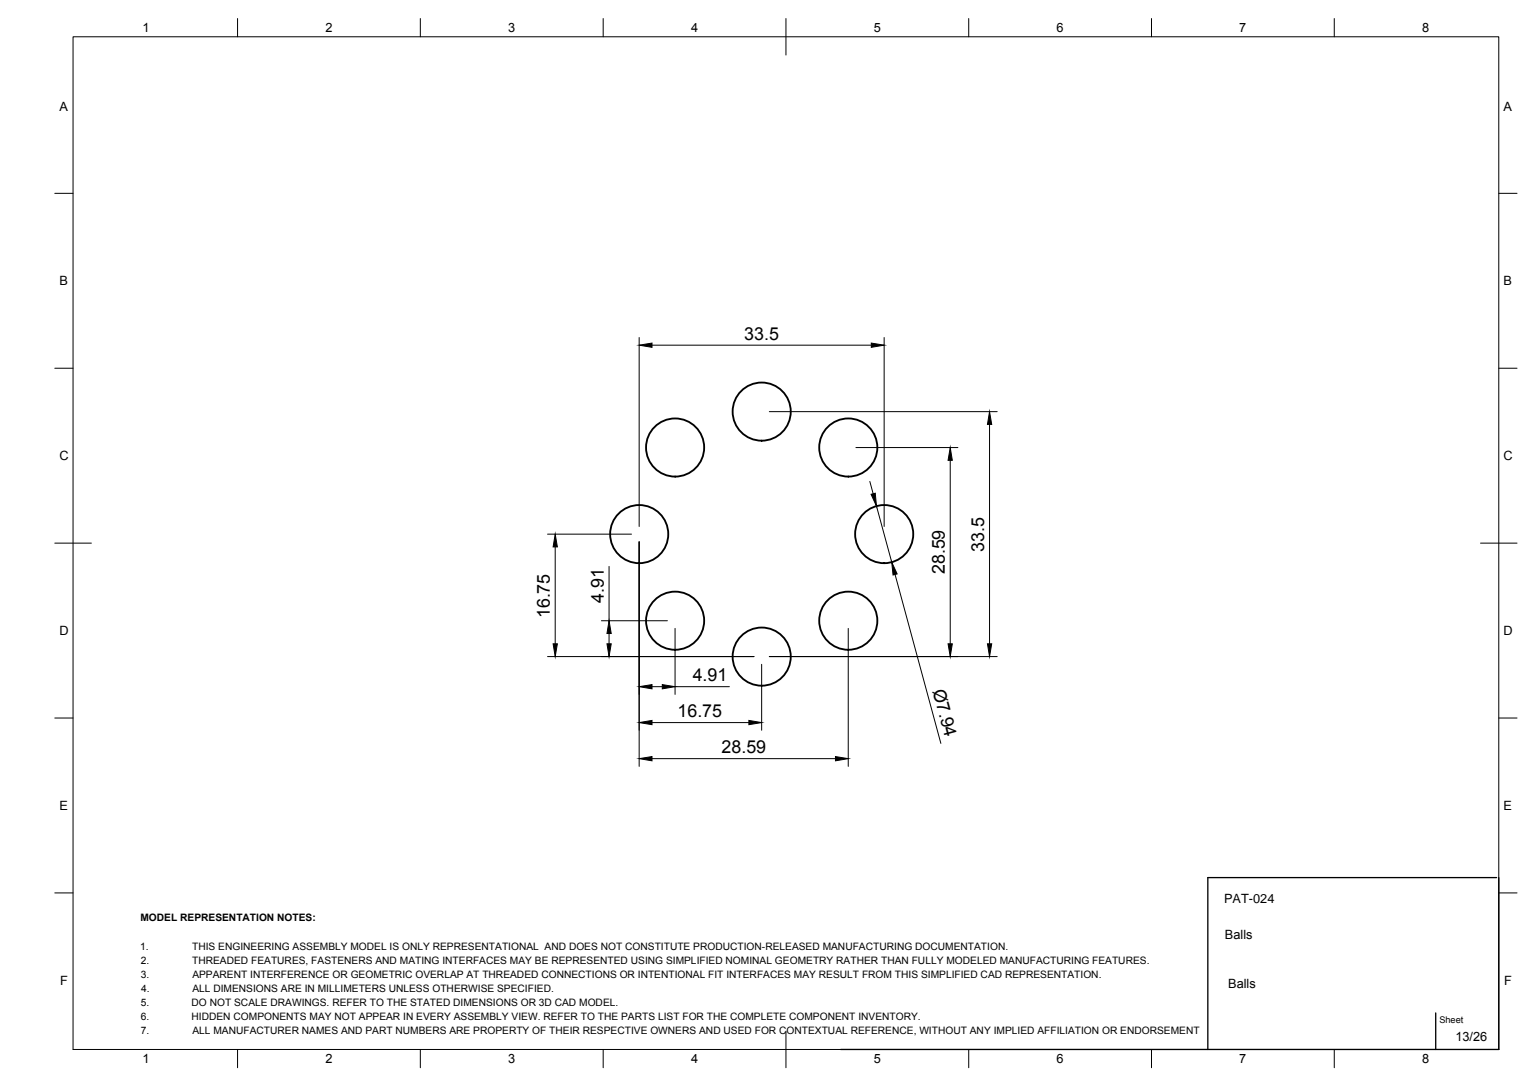
ISO-10303-21;
HEADER;
/* Generated by software containing ST-Developer
 * from STEP Tools, Inc. (www.steptools.com) 
 */

FILE_DESCRIPTION(
/* description */ ('Compact handwheel screw vise'),
/* implementation_level */ '2;1');

FILE_NAME(
/* name */ 'Balls.step',
/* time_stamp */ '2026-10-29T16:08:22-07:00',
/* author */ (''),
/* organization */ (''),
/* preprocessor_version */ 'ST-DEVELOPER v20.2',
/* originating_system */ 'Autodesk Translation Framework v15.17.0.0',
/* authorisation */ '');

FILE_SCHEMA (('AUTOMOTIVE_DESIGN { 1 0 10303 214 3 1 1 }'));
ENDSEC;

DATA;
#10=MECHANICAL_DESIGN_GEOMETRIC_PRESENTATION_REPRESENTATION('',(#653,#654,#655,#656,#657,#658,#659,#660),#25074);
#541=SPHERICAL_SURFACE('',#8614,0.3969);
#542=SPHERICAL_SURFACE('',#8616,0.3969);
#543=SPHERICAL_SURFACE('',#8618,0.3969);
#544=SPHERICAL_SURFACE('',#8620,0.3969);
#545=SPHERICAL_SURFACE('',#8622,0.3969);
#546=SPHERICAL_SURFACE('',#8624,0.3969);
#547=SPHERICAL_SURFACE('',#8626,0.3969);
#548=SPHERICAL_SURFACE('',#8628,0.3969);
#597=SHAPE_REPRESENTATION_RELATIONSHIP('SRR','None',#25206,#625);
#625=ADVANCED_BREP_SHAPE_REPRESENTATION('',(#688,#689,#690,#691,#692,#693,
#694,#695),#25053);
#653=STYLED_ITEM('',(#25439),#688);
#654=STYLED_ITEM('',(#25439),#689);
#655=STYLED_ITEM('',(#25439),#690);
#656=STYLED_ITEM('',(#25439),#691);
#657=STYLED_ITEM('',(#25439),#692);
#658=STYLED_ITEM('',(#25439),#693);
#659=STYLED_ITEM('',(#25439),#694);
#660=STYLED_ITEM('',(#25439),#695);
#688=MANIFOLD_SOLID_BREP('Body1',#8062);
#689=MANIFOLD_SOLID_BREP('Body2',#8063);
#690=MANIFOLD_SOLID_BREP('Body3',#8064);
#691=MANIFOLD_SOLID_BREP('Body4',#8065);
#692=MANIFOLD_SOLID_BREP('Body5',#8066);
#693=MANIFOLD_SOLID_BREP('Body6',#8067);
#694=MANIFOLD_SOLID_BREP('Body7',#8068);
#695=MANIFOLD_SOLID_BREP('Body8',#8069);
#1121=FACE_OUTER_BOUND('',#1643,.T.);
#1122=FACE_OUTER_BOUND('',#1644,.T.);
#1123=FACE_OUTER_BOUND('',#1645,.T.);
#1124=FACE_OUTER_BOUND('',#1646,.T.);
#1125=FACE_OUTER_BOUND('',#1647,.T.);
#1126=FACE_OUTER_BOUND('',#1648,.T.);
#1127=FACE_OUTER_BOUND('',#1649,.T.);
#1128=FACE_OUTER_BOUND('',#1650,.T.);
#1643=EDGE_LOOP('',(#5595,#5596));
#1644=EDGE_LOOP('',(#5597,#5598));
#1645=EDGE_LOOP('',(#5599,#5600));
#1646=EDGE_LOOP('',(#5601,#5602));
#1647=EDGE_LOOP('',(#5603,#5604));
#1648=EDGE_LOOP('',(#5605,#5606));
#1649=EDGE_LOOP('',(#5607,#5608));
#1650=EDGE_LOOP('',(#5609,#5610));
#3169=CIRCLE('',#8615,0.3969);
#3170=CIRCLE('',#8617,0.3969);
#3171=CIRCLE('',#8619,0.3969);
#3172=CIRCLE('',#8621,0.3969);
#3173=CIRCLE('',#8623,0.3969);
#3174=CIRCLE('',#8625,0.3969);
#3175=CIRCLE('',#8627,0.3969);
#3176=CIRCLE('',#8629,0.3969);
#3476=VERTEX_POINT('',#11802);
#3477=VERTEX_POINT('',#11803);
#3478=VERTEX_POINT('',#11806);
#3479=VERTEX_POINT('',#11807);
#3480=VERTEX_POINT('',#11810);
#3481=VERTEX_POINT('',#11811);
#3482=VERTEX_POINT('',#11814);
#3483=VERTEX_POINT('',#11815);
#3484=VERTEX_POINT('',#11818);
#3485=VERTEX_POINT('',#11819);
#3486=VERTEX_POINT('',#11822);
#3487=VERTEX_POINT('',#11823);
#3488=VERTEX_POINT('',#11826);
#3489=VERTEX_POINT('',#11827);
#3490=VERTEX_POINT('',#11830);
#3491=VERTEX_POINT('',#11831);
#4284=EDGE_CURVE('',#3476,#3477,#3169,.T.);
#4285=EDGE_CURVE('',#3478,#3479,#3170,.T.);
#4286=EDGE_CURVE('',#3480,#3481,#3171,.T.);
#4287=EDGE_CURVE('',#3482,#3483,#3172,.T.);
#4288=EDGE_CURVE('',#3484,#3485,#3173,.T.);
#4289=EDGE_CURVE('',#3486,#3487,#3174,.T.);
#4290=EDGE_CURVE('',#3488,#3489,#3175,.T.);
#4291=EDGE_CURVE('',#3490,#3491,#3176,.T.);
#5595=ORIENTED_EDGE('',*,*,#4284,.T.);
#5596=ORIENTED_EDGE('',*,*,#4284,.F.);
#5597=ORIENTED_EDGE('',*,*,#4285,.T.);
#5598=ORIENTED_EDGE('',*,*,#4285,.F.);
#5599=ORIENTED_EDGE('',*,*,#4286,.T.);
#5600=ORIENTED_EDGE('',*,*,#4286,.F.);
#5601=ORIENTED_EDGE('',*,*,#4287,.T.);
#5602=ORIENTED_EDGE('',*,*,#4287,.F.);
#5603=ORIENTED_EDGE('',*,*,#4288,.T.);
#5604=ORIENTED_EDGE('',*,*,#4288,.F.);
#5605=ORIENTED_EDGE('',*,*,#4289,.T.);
#5606=ORIENTED_EDGE('',*,*,#4289,.F.);
#5607=ORIENTED_EDGE('',*,*,#4290,.T.);
#5608=ORIENTED_EDGE('',*,*,#4290,.F.);
#5609=ORIENTED_EDGE('',*,*,#4291,.T.);
#5610=ORIENTED_EDGE('',*,*,#4291,.F.);
#7691=ADVANCED_FACE('',(#1121),#541,.T.);
#7692=ADVANCED_FACE('',(#1122),#542,.T.);
#7693=ADVANCED_FACE('',(#1123),#543,.T.);
#7694=ADVANCED_FACE('',(#1124),#544,.T.);
#7695=ADVANCED_FACE('',(#1125),#545,.T.);
#7696=ADVANCED_FACE('',(#1126),#546,.T.);
#7697=ADVANCED_FACE('',(#1127),#547,.T.);
#7698=ADVANCED_FACE('',(#1128),#548,.T.);
#8062=CLOSED_SHELL('',(#7691));
#8063=CLOSED_SHELL('',(#7692));
#8064=CLOSED_SHELL('',(#7693));
#8065=CLOSED_SHELL('',(#7694));
#8066=CLOSED_SHELL('',(#7695));
#8067=CLOSED_SHELL('',(#7696));
#8068=CLOSED_SHELL('',(#7697));
#8069=CLOSED_SHELL('',(#7698));
#8613=AXIS2_PLACEMENT_3D('',#11800,#9755,#9756);
#8614=AXIS2_PLACEMENT_3D('',#11801,#9757,#9758);
#8615=AXIS2_PLACEMENT_3D('',#11804,#9759,#9760);
#8616=AXIS2_PLACEMENT_3D('',#11805,#9761,#9762);
#8617=AXIS2_PLACEMENT_3D('',#11808,#9763,#9764);
#8618=AXIS2_PLACEMENT_3D('',#11809,#9765,#9766);
#8619=AXIS2_PLACEMENT_3D('',#11812,#9767,#9768);
#8620=AXIS2_PLACEMENT_3D('',#11813,#9769,#9770);
#8621=AXIS2_PLACEMENT_3D('',#11816,#9771,#9772);
#8622=AXIS2_PLACEMENT_3D('',#11817,#9773,#9774);
#8623=AXIS2_PLACEMENT_3D('',#11820,#9775,#9776);
#8624=AXIS2_PLACEMENT_3D('',#11821,#9777,#9778);
#8625=AXIS2_PLACEMENT_3D('',#11824,#9779,#9780);
#8626=AXIS2_PLACEMENT_3D('',#11825,#9781,#9782);
#8627=AXIS2_PLACEMENT_3D('',#11828,#9783,#9784);
#8628=AXIS2_PLACEMENT_3D('',#11829,#9785,#9786);
#8629=AXIS2_PLACEMENT_3D('',#11832,#9787,#9788);
#9755=DIRECTION('axis',(0.,0.,1.));
#9756=DIRECTION('refdir',(1.,0.,0.));
#9757=DIRECTION('center_axis',(0.,0.,1.));
#9758=DIRECTION('ref_axis',(1.,0.,0.));
#9759=DIRECTION('center_axis',(1.22464679914735E-16,-1.,0.));
#9760=DIRECTION('ref_axis',(-1.,-1.22464679914735E-16,0.));
#9761=DIRECTION('center_axis',(0.707106781186548,0.,0.707106781186548));
#9762=DIRECTION('ref_axis',(0.707106781186548,0.,-0.707106781186548));
#9763=DIRECTION('center_axis',(8.65956056235493E-17,-1.,-8.65956056235493E-17));
#9764=DIRECTION('ref_axis',(-0.707106781186548,-1.22464679914735E-16,0.707106781186548));
#9765=DIRECTION('center_axis',(1.,0.,0.));
#9766=DIRECTION('ref_axis',(6.12323399573677E-17,0.,-1.));
#9767=DIRECTION('center_axis',(7.49879891330929E-33,-1.,-1.22464679914735E-16));
#9768=DIRECTION('ref_axis',(-6.12323399573677E-17,-1.22464679914735E-16,
1.));
#9769=DIRECTION('center_axis',(0.707106781186548,0.,-0.707106781186548));
#9770=DIRECTION('ref_axis',(-0.707106781186548,0.,-0.707106781186548));
#9771=DIRECTION('center_axis',(-8.65956056235493E-17,-1.,-8.65956056235493E-17));
#9772=DIRECTION('ref_axis',(0.707106781186548,-1.22464679914735E-16,0.707106781186548));
#9773=DIRECTION('center_axis',(0.,0.,-1.));
#9774=DIRECTION('ref_axis',(-1.,0.,-1.22464679914735E-16));
#9775=DIRECTION('center_axis',(-1.22464679914735E-16,-1.,-1.49975978266186E-32));
#9776=DIRECTION('ref_axis',(1.,-1.22464679914735E-16,1.22464679914735E-16));
#9777=DIRECTION('center_axis',(-0.707106781186548,0.,-0.707106781186548));
#9778=DIRECTION('ref_axis',(-0.707106781186548,0.,0.707106781186548));
#9779=DIRECTION('center_axis',(-8.65956056235493E-17,-1.,8.65956056235493E-17));
#9780=DIRECTION('ref_axis',(0.707106781186548,-1.22464679914735E-16,-0.707106781186548));
#9781=DIRECTION('center_axis',(-1.,0.,0.));
#9782=DIRECTION('ref_axis',(-1.83697019872103E-16,0.,1.));
#9783=DIRECTION('center_axis',(-2.24963967399279E-32,-1.,1.22464679914735E-16));
#9784=DIRECTION('ref_axis',(1.83697019872103E-16,-1.22464679914735E-16,
-1.));
#9785=DIRECTION('center_axis',(-0.707106781186548,0.,0.707106781186548));
#9786=DIRECTION('ref_axis',(0.707106781186548,0.,0.707106781186548));
#9787=DIRECTION('center_axis',(8.65956056235493E-17,-1.,8.65956056235494E-17));
#9788=DIRECTION('ref_axis',(-0.707106781186548,-1.22464679914735E-16,-0.707106781186548));
#11800=CARTESIAN_POINT('',(0.,0.,0.));
#11801=CARTESIAN_POINT('Origin',(1.675,0.,0.));
#11802=CARTESIAN_POINT('',(1.675,-2.97627328869245E-33,0.3969));
#11803=CARTESIAN_POINT('',(1.675,-2.97627328869245E-33,-0.3969));
#11804=CARTESIAN_POINT('Origin',(1.675,0.,0.));
#11805=CARTESIAN_POINT('Origin',(1.18440385848747,0.,-1.18440385848747));
#11806=CARTESIAN_POINT('',(1.46505453994041,3.1867025333467E-33,-0.903753177034526));
#11807=CARTESIAN_POINT('',(0.903753177034527,-9.13924911073161E-33,-1.46505453994041));
#11808=CARTESIAN_POINT('Origin',(1.18440385848747,0.,-1.18440385848747));
#11809=CARTESIAN_POINT('Origin',(1.02564169428591E-16,0.,-1.675));
#11810=CARTESIAN_POINT('',(0.3969,-2.97627328869246E-33,-1.675));
#11811=CARTESIAN_POINT('',(-0.3969,-2.97627328869245E-33,-1.675));
#11812=CARTESIAN_POINT('Origin',(1.02564169428591E-16,0.,-1.675));
#11813=CARTESIAN_POINT('Origin',(-1.18440385848747,0.,-1.18440385848747));
#11814=CARTESIAN_POINT('',(-0.903753177034526,3.1867025333467E-33,-1.46505453994041));
#11815=CARTESIAN_POINT('',(-1.46505453994041,-9.13924911073161E-33,-0.903753177034527));
#11816=CARTESIAN_POINT('Origin',(-1.18440385848747,0.,-1.18440385848747));
#11817=CARTESIAN_POINT('Origin',(-1.675,0.,-2.05128338857182E-16));
#11818=CARTESIAN_POINT('',(-1.675,-2.97627328869246E-33,-0.3969));
#11819=CARTESIAN_POINT('',(-1.675,-2.97627328869245E-33,0.3969));
#11820=CARTESIAN_POINT('Origin',(-1.675,0.,-2.05128338857182E-16));
#11821=CARTESIAN_POINT('Origin',(-1.18440385848747,0.,1.18440385848747));
#11822=CARTESIAN_POINT('',(-1.46505453994041,6.26819044436628E-33,0.903753177034526));
#11823=CARTESIAN_POINT('',(-0.903753177034527,-1.22207370217512E-32,1.46505453994041));
#11824=CARTESIAN_POINT('Origin',(-1.18440385848747,0.,1.18440385848747));
#11825=CARTESIAN_POINT('Origin',(-3.07692508285772E-16,0.,1.675));
#11826=CARTESIAN_POINT('',(-0.3969,-2.97627328869246E-33,1.675));
#11827=CARTESIAN_POINT('',(0.396899999999999,-2.97627328869245E-33,1.675));
#11828=CARTESIAN_POINT('Origin',(-3.07692508285772E-16,0.,1.675));
#11829=CARTESIAN_POINT('Origin',(1.18440385848747,0.,1.18440385848747));
#11830=CARTESIAN_POINT('',(0.903753177034526,9.34967835538585E-33,1.46505453994041));
#11831=CARTESIAN_POINT('',(1.46505453994041,-1.53022249327708E-32,0.903753177034527));
#11832=CARTESIAN_POINT('Origin',(1.18440385848747,0.,1.18440385848747));
#25019=UNCERTAINTY_MEASURE_WITH_UNIT(LENGTH_MEASURE(0.001),#25075,
'DISTANCE_ACCURACY_VALUE',
'Maximum model space distance between geometric entities at asserted c
onnectivities');
#25040=UNCERTAINTY_MEASURE_WITH_UNIT(LENGTH_MEASURE(0.001),#25075,
'DISTANCE_ACCURACY_VALUE',
'Maximum model space distance between geometric entities at asserted c
onnectivities');
#25053=(
GEOMETRIC_REPRESENTATION_CONTEXT(3)
GLOBAL_UNCERTAINTY_ASSIGNED_CONTEXT((#25019))
GLOBAL_UNIT_ASSIGNED_CONTEXT((#25075,#25077,#25078))
REPRESENTATION_CONTEXT('','3D')
);
#25074=(
GEOMETRIC_REPRESENTATION_CONTEXT(3)
GLOBAL_UNCERTAINTY_ASSIGNED_CONTEXT((#25040))
GLOBAL_UNIT_ASSIGNED_CONTEXT((#25075,#25077,#25078))
REPRESENTATION_CONTEXT('','3D')
);
#25075=(
LENGTH_UNIT()
NAMED_UNIT(*)
SI_UNIT(.CENTI.,.METRE.)
);
#25077=(
NAMED_UNIT(*)
PLANE_ANGLE_UNIT()
SI_UNIT($,.RADIAN.)
);
#25078=(
NAMED_UNIT(*)
SI_UNIT($,.STERADIAN.)
SOLID_ANGLE_UNIT()
);
#25091=SHAPE_DEFINITION_REPRESENTATION(#25124,#25206);
#25124=PRODUCT_DEFINITION_SHAPE('',$,#25240);
#25206=SHAPE_REPRESENTATION('',(#8613),#25053);
#25227=PRODUCT_DEFINITION_CONTEXT('part definition',#25328,'design');
#25240=PRODUCT_DEFINITION('Balls','Balls',#25273,#25227);
#25273=PRODUCT_DEFINITION_FORMATION('',$,#25342);
#25328=APPLICATION_CONTEXT(
'Core Data for Automotive Mechanical Design Process');
#25329=PRODUCT_CONTEXT('part definition',#25328,'mechanical');
#25342=PRODUCT('Balls','Balls','Balls',(#25329));
#25433=COLOUR_RGB('Grey',0.48,0.52,0.57);
#25434=FILL_AREA_STYLE_COLOUR('',#25433);
#25435=FILL_AREA_STYLE('',(#25434));
#25436=SURFACE_STYLE_FILL_AREA(#25435);
#25437=SURFACE_SIDE_STYLE('',(#25436));
#25438=SURFACE_STYLE_USAGE(.BOTH.,#25437);
#25439=PRESENTATION_STYLE_ASSIGNMENT((#25438));
ENDSEC;
END-ISO-10303-21;
